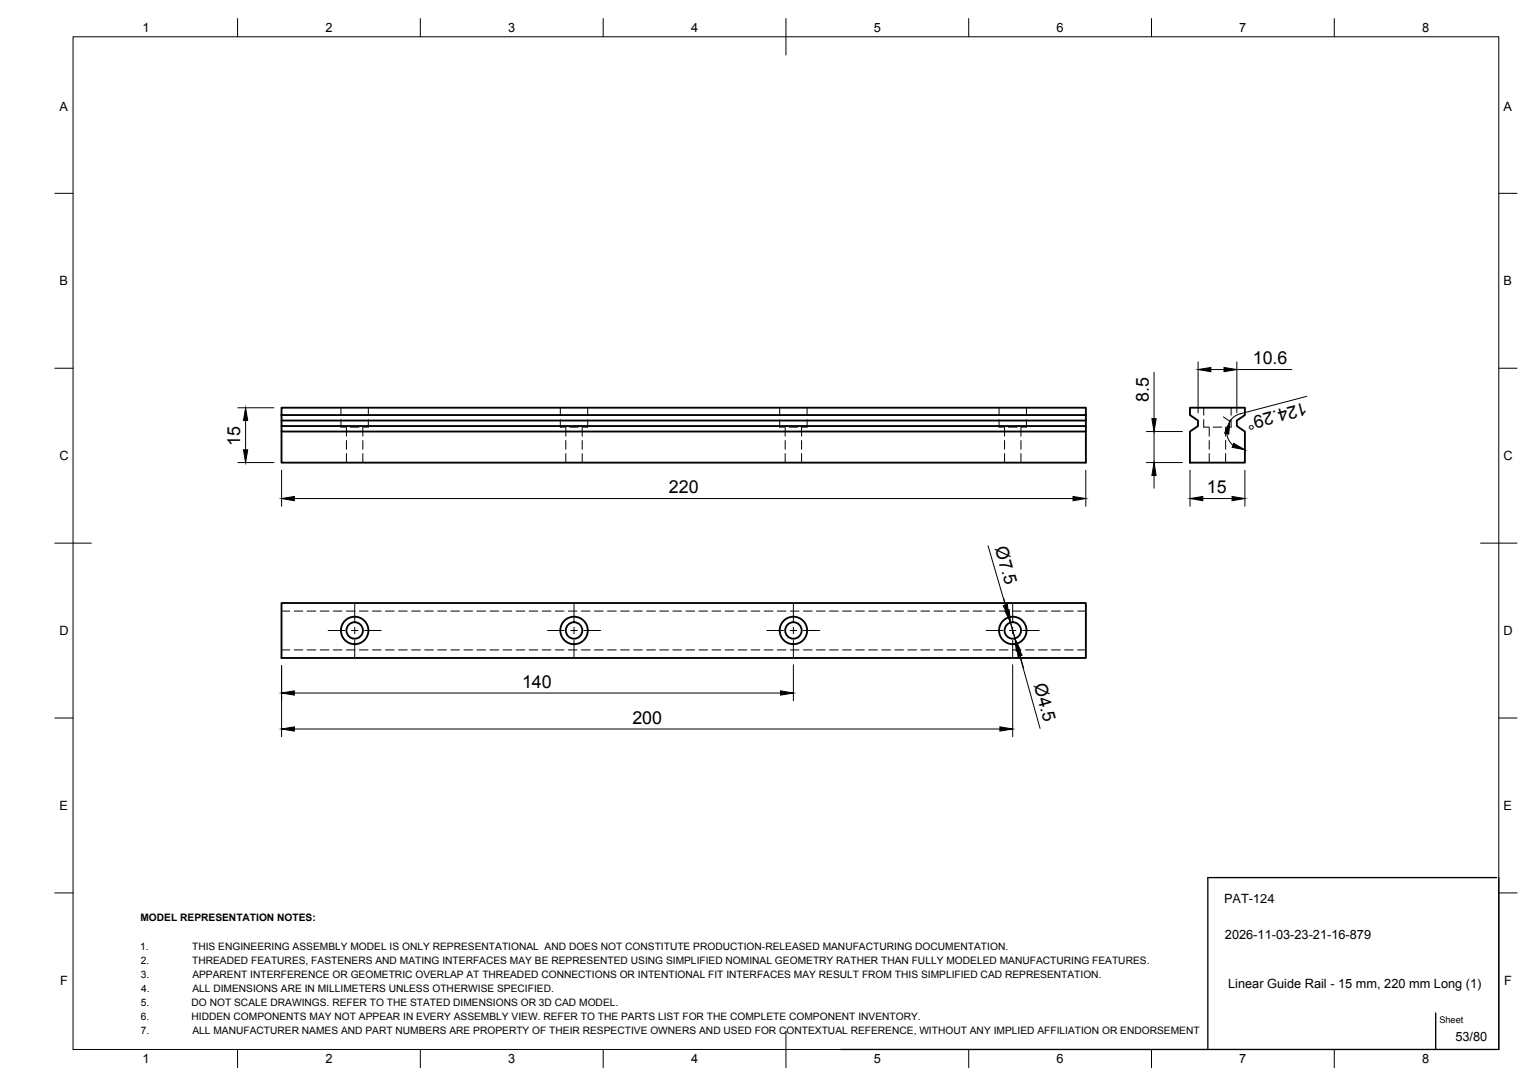
ISO-10303-21;
HEADER;
/* Generated by software containing ST-Developer
 * from STEP Tools, Inc. (www.steptools.com) 
 */

FILE_DESCRIPTION(
/* description */ ('XY cross-slide table'),
/* implementation_level */ '2;1');

FILE_NAME(
/* name */ 'Linear Guide Rail - 15 mm, 220 mm Long (1).step',
/* time_stamp */ '2026-10-28T03:22:46-07:00',
/* author */ (''),
/* organization */ (''),
/* preprocessor_version */ 'ST-DEVELOPER v20.2',
/* originating_system */ 'Autodesk Translation Framework v15.17.0.0',
/* authorisation */ '');

FILE_SCHEMA (('AUTOMOTIVE_DESIGN { 1 0 10303 214 3 1 1 }'));
ENDSEC;

DATA;
#10=MECHANICAL_DESIGN_GEOMETRIC_PRESENTATION_REPRESENTATION('',(#1735),#62984);
#1554=SHAPE_REPRESENTATION_RELATIONSHIP('SRR','None',#63409,#1637);
#1637=ADVANCED_BREP_SHAPE_REPRESENTATION('',(#1844),#62946);
#1735=STYLED_ITEM('',(#63905),#1844);
#1844=MANIFOLD_SOLID_BREP('Body1',#23033);
#2189=FACE_BOUND('',#5267,.T.);
#2190=FACE_BOUND('',#5270,.T.);
#2191=FACE_BOUND('',#5273,.T.);
#2192=FACE_BOUND('',#5276,.T.);
#2193=FACE_BOUND('',#5286,.T.);
#2194=FACE_BOUND('',#5287,.T.);
#2195=FACE_BOUND('',#5288,.T.);
#2196=FACE_BOUND('',#5289,.T.);
#2197=FACE_BOUND('',#5296,.T.);
#2198=FACE_BOUND('',#5297,.T.);
#2199=FACE_BOUND('',#5298,.T.);
#2200=FACE_BOUND('',#5299,.T.);
#2644=PLANE('',#25491);
#2645=PLANE('',#25496);
#2646=PLANE('',#25501);
#2647=PLANE('',#25506);
#2648=PLANE('',#25516);
#2649=PLANE('',#25517);
#2650=PLANE('',#25518);
#2651=PLANE('',#25519);
#2652=PLANE('',#25520);
#2653=PLANE('',#25521);
#2654=PLANE('',#25522);
#2655=PLANE('',#25523);
#2656=PLANE('',#25524);
#2657=PLANE('',#25525);
#2658=PLANE('',#25526);
#2659=PLANE('',#25527);
#2660=PLANE('',#25528);
#2661=PLANE('',#25529);
#3649=FACE_OUTER_BOUND('',#5265,.T.);
#3650=FACE_OUTER_BOUND('',#5266,.T.);
#3651=FACE_OUTER_BOUND('',#5268,.T.);
#3652=FACE_OUTER_BOUND('',#5269,.T.);
#3653=FACE_OUTER_BOUND('',#5271,.T.);
#3654=FACE_OUTER_BOUND('',#5272,.T.);
#3655=FACE_OUTER_BOUND('',#5274,.T.);
#3656=FACE_OUTER_BOUND('',#5275,.T.);
#3657=FACE_OUTER_BOUND('',#5277,.T.);
#3658=FACE_OUTER_BOUND('',#5278,.T.);
#3659=FACE_OUTER_BOUND('',#5279,.T.);
#3660=FACE_OUTER_BOUND('',#5280,.T.);
#3661=FACE_OUTER_BOUND('',#5281,.T.);
#3662=FACE_OUTER_BOUND('',#5282,.T.);
#3663=FACE_OUTER_BOUND('',#5283,.T.);
#3664=FACE_OUTER_BOUND('',#5284,.T.);
#3665=FACE_OUTER_BOUND('',#5285,.T.);
#3666=FACE_OUTER_BOUND('',#5290,.T.);
#3667=FACE_OUTER_BOUND('',#5291,.T.);
#3668=FACE_OUTER_BOUND('',#5292,.T.);
#3669=FACE_OUTER_BOUND('',#5293,.T.);
#3670=FACE_OUTER_BOUND('',#5294,.T.);
#3671=FACE_OUTER_BOUND('',#5295,.T.);
#3672=FACE_OUTER_BOUND('',#5300,.T.);
#3673=FACE_OUTER_BOUND('',#5301,.T.);
#3674=FACE_OUTER_BOUND('',#5302,.T.);
#5265=EDGE_LOOP('',(#18508,#18509,#18510,#18511));
#5266=EDGE_LOOP('',(#18512));
#5267=EDGE_LOOP('',(#18513));
#5268=EDGE_LOOP('',(#18514,#18515,#18516,#18517));
#5269=EDGE_LOOP('',(#18518));
#5270=EDGE_LOOP('',(#18519));
#5271=EDGE_LOOP('',(#18520,#18521,#18522,#18523));
#5272=EDGE_LOOP('',(#18524));
#5273=EDGE_LOOP('',(#18525));
#5274=EDGE_LOOP('',(#18526,#18527,#18528,#18529));
#5275=EDGE_LOOP('',(#18530));
#5276=EDGE_LOOP('',(#18531));
#5277=EDGE_LOOP('',(#18532,#18533,#18534,#18535));
#5278=EDGE_LOOP('',(#18536,#18537,#18538,#18539));
#5279=EDGE_LOOP('',(#18540,#18541,#18542,#18543));
#5280=EDGE_LOOP('',(#18544,#18545,#18546,#18547));
#5281=EDGE_LOOP('',(#18548,#18549,#18550,#18551));
#5282=EDGE_LOOP('',(#18552,#18553,#18554,#18555));
#5283=EDGE_LOOP('',(#18556,#18557,#18558,#18559));
#5284=EDGE_LOOP('',(#18560,#18561,#18562,#18563));
#5285=EDGE_LOOP('',(#18564,#18565,#18566,#18567));
#5286=EDGE_LOOP('',(#18568));
#5287=EDGE_LOOP('',(#18569));
#5288=EDGE_LOOP('',(#18570));
#5289=EDGE_LOOP('',(#18571));
#5290=EDGE_LOOP('',(#18572,#18573,#18574,#18575));
#5291=EDGE_LOOP('',(#18576,#18577,#18578,#18579));
#5292=EDGE_LOOP('',(#18580,#18581,#18582,#18583));
#5293=EDGE_LOOP('',(#18584,#18585,#18586,#18587));
#5294=EDGE_LOOP('',(#18588,#18589,#18590,#18591));
#5295=EDGE_LOOP('',(#18592,#18593,#18594,#18595));
#5296=EDGE_LOOP('',(#18596));
#5297=EDGE_LOOP('',(#18597));
#5298=EDGE_LOOP('',(#18598));
#5299=EDGE_LOOP('',(#18599));
#5300=EDGE_LOOP('',(#18600,#18601,#18602,#18603));
#5301=EDGE_LOOP('',(#18604,#18605,#18606,#18607,#18608,#18609,#18610,#18611,
#18612,#18613,#18614,#18615));
#5302=EDGE_LOOP('',(#18616,#18617,#18618,#18619,#18620,#18621,#18622,#18623,
#18624,#18625,#18626,#18627));
#6793=LINE('',#48410,#8280);
#6794=LINE('',#48419,#8281);
#6795=LINE('',#48428,#8282);
#6796=LINE('',#48437,#8283);
#6797=LINE('',#48445,#8284);
#6798=LINE('',#48449,#8285);
#6799=LINE('',#48453,#8286);
#6800=LINE('',#48457,#8287);
#6801=LINE('',#48461,#8288);
#6802=LINE('',#48463,#8289);
#6803=LINE('',#48465,#8290);
#6804=LINE('',#48466,#8291);
#6805=LINE('',#48469,#8292);
#6806=LINE('',#48471,#8293);
#6807=LINE('',#48472,#8294);
#6808=LINE('',#48475,#8295);
#6809=LINE('',#48477,#8296);
#6810=LINE('',#48478,#8297);
#6811=LINE('',#48481,#8298);
#6812=LINE('',#48483,#8299);
#6813=LINE('',#48484,#8300);
#6814=LINE('',#48487,#8301);
#6815=LINE('',#48489,#8302);
#6816=LINE('',#48490,#8303);
#6817=LINE('',#48493,#8304);
#6818=LINE('',#48495,#8305);
#6819=LINE('',#48496,#8306);
#6820=LINE('',#48499,#8307);
#6821=LINE('',#48501,#8308);
#6822=LINE('',#48502,#8309);
#6823=LINE('',#48505,#8310);
#6824=LINE('',#48507,#8311);
#6825=LINE('',#48508,#8312);
#6826=LINE('',#48511,#8313);
#6827=LINE('',#48513,#8314);
#6828=LINE('',#48514,#8315);
#6829=LINE('',#48517,#8316);
#6830=LINE('',#48519,#8317);
#6831=LINE('',#48520,#8318);
#6832=LINE('',#48523,#8319);
#6833=LINE('',#48525,#8320);
#6834=LINE('',#48526,#8321);
#6835=LINE('',#48528,#8322);
#6836=LINE('',#48529,#8323);
#8280=VECTOR('',#30328,0.375);
#8281=VECTOR('',#30339,0.375);
#8282=VECTOR('',#30350,0.375);
#8283=VECTOR('',#30361,0.375);
#8284=VECTOR('',#30372,0.225);
#8285=VECTOR('',#30377,0.225);
#8286=VECTOR('',#30382,0.225);
#8287=VECTOR('',#30387,0.225000000000001);
#8288=VECTOR('',#30390,1.);
#8289=VECTOR('',#30391,1.);
#8290=VECTOR('',#30392,1.);
#8291=VECTOR('',#30393,1.);
#8292=VECTOR('',#30396,1.);
#8293=VECTOR('',#30397,1.);
#8294=VECTOR('',#30398,1.);
#8295=VECTOR('',#30401,1.);
#8296=VECTOR('',#30402,1.);
#8297=VECTOR('',#30403,1.);
#8298=VECTOR('',#30406,1.);
#8299=VECTOR('',#30407,1.);
#8300=VECTOR('',#30408,1.);
#8301=VECTOR('',#30411,1.);
#8302=VECTOR('',#30412,1.);
#8303=VECTOR('',#30413,1.);
#8304=VECTOR('',#30416,1.);
#8305=VECTOR('',#30417,1.);
#8306=VECTOR('',#30418,1.);
#8307=VECTOR('',#30421,1.);
#8308=VECTOR('',#30422,1.);
#8309=VECTOR('',#30423,1.);
#8310=VECTOR('',#30426,1.);
#8311=VECTOR('',#30427,1.);
#8312=VECTOR('',#30428,1.);
#8313=VECTOR('',#30431,1.);
#8314=VECTOR('',#30432,1.);
#8315=VECTOR('',#30433,1.);
#8316=VECTOR('',#30436,1.);
#8317=VECTOR('',#30437,1.);
#8318=VECTOR('',#30438,1.);
#8319=VECTOR('',#30441,1.);
#8320=VECTOR('',#30442,1.);
#8321=VECTOR('',#30443,1.);
#8322=VECTOR('',#30446,1.);
#8323=VECTOR('',#30447,1.);
#9451=CIRCLE('',#25489,0.375);
#9452=CIRCLE('',#25490,0.375);
#9453=CIRCLE('',#25492,0.225);
#9454=CIRCLE('',#25494,0.375);
#9455=CIRCLE('',#25495,0.375);
#9456=CIRCLE('',#25497,0.225);
#9457=CIRCLE('',#25499,0.375);
#9458=CIRCLE('',#25500,0.375);
#9459=CIRCLE('',#25502,0.225);
#9460=CIRCLE('',#25504,0.375);
#9461=CIRCLE('',#25505,0.375);
#9462=CIRCLE('',#25507,0.225000000000001);
#9463=CIRCLE('',#25509,0.225);
#9464=CIRCLE('',#25511,0.225);
#9465=CIRCLE('',#25513,0.225);
#9466=CIRCLE('',#25515,0.225000000000001);
#10981=VERTEX_POINT('',#48407);
#10982=VERTEX_POINT('',#48409);
#10983=VERTEX_POINT('',#48413);
#10984=VERTEX_POINT('',#48416);
#10985=VERTEX_POINT('',#48418);
#10986=VERTEX_POINT('',#48422);
#10987=VERTEX_POINT('',#48425);
#10988=VERTEX_POINT('',#48427);
#10989=VERTEX_POINT('',#48431);
#10990=VERTEX_POINT('',#48434);
#10991=VERTEX_POINT('',#48436);
#10992=VERTEX_POINT('',#48440);
#10993=VERTEX_POINT('',#48443);
#10994=VERTEX_POINT('',#48447);
#10995=VERTEX_POINT('',#48451);
#10996=VERTEX_POINT('',#48455);
#10997=VERTEX_POINT('',#48459);
#10998=VERTEX_POINT('',#48460);
#10999=VERTEX_POINT('',#48462);
#11000=VERTEX_POINT('',#48464);
#11001=VERTEX_POINT('',#48468);
#11002=VERTEX_POINT('',#48470);
#11003=VERTEX_POINT('',#48474);
#11004=VERTEX_POINT('',#48476);
#11005=VERTEX_POINT('',#48480);
#11006=VERTEX_POINT('',#48482);
#11007=VERTEX_POINT('',#48486);
#11008=VERTEX_POINT('',#48488);
#11009=VERTEX_POINT('',#48492);
#11010=VERTEX_POINT('',#48494);
#11011=VERTEX_POINT('',#48498);
#11012=VERTEX_POINT('',#48500);
#11013=VERTEX_POINT('',#48504);
#11014=VERTEX_POINT('',#48506);
#11015=VERTEX_POINT('',#48510);
#11016=VERTEX_POINT('',#48512);
#11017=VERTEX_POINT('',#48516);
#11018=VERTEX_POINT('',#48518);
#11019=VERTEX_POINT('',#48522);
#11020=VERTEX_POINT('',#48524);
#13638=EDGE_CURVE('',#10981,#10981,#9451,.T.);
#13639=EDGE_CURVE('',#10981,#10982,#6793,.T.);
#13640=EDGE_CURVE('',#10982,#10982,#9452,.T.);
#13641=EDGE_CURVE('',#10983,#10983,#9453,.T.);
#13642=EDGE_CURVE('',#10984,#10984,#9454,.T.);
#13643=EDGE_CURVE('',#10984,#10985,#6794,.T.);
#13644=EDGE_CURVE('',#10985,#10985,#9455,.T.);
#13645=EDGE_CURVE('',#10986,#10986,#9456,.T.);
#13646=EDGE_CURVE('',#10987,#10987,#9457,.T.);
#13647=EDGE_CURVE('',#10987,#10988,#6795,.T.);
#13648=EDGE_CURVE('',#10988,#10988,#9458,.T.);
#13649=EDGE_CURVE('',#10989,#10989,#9459,.T.);
#13650=EDGE_CURVE('',#10990,#10990,#9460,.T.);
#13651=EDGE_CURVE('',#10990,#10991,#6796,.T.);
#13652=EDGE_CURVE('',#10991,#10991,#9461,.T.);
#13653=EDGE_CURVE('',#10992,#10992,#9462,.T.);
#13654=EDGE_CURVE('',#10993,#10993,#9463,.T.);
#13655=EDGE_CURVE('',#10993,#10983,#6797,.T.);
#13656=EDGE_CURVE('',#10994,#10994,#9464,.T.);
#13657=EDGE_CURVE('',#10994,#10986,#6798,.T.);
#13658=EDGE_CURVE('',#10995,#10995,#9465,.T.);
#13659=EDGE_CURVE('',#10995,#10989,#6799,.T.);
#13660=EDGE_CURVE('',#10996,#10996,#9466,.T.);
#13661=EDGE_CURVE('',#10996,#10992,#6800,.T.);
#13662=EDGE_CURVE('',#10997,#10998,#6801,.T.);
#13663=EDGE_CURVE('',#10998,#10999,#6802,.T.);
#13664=EDGE_CURVE('',#11000,#10999,#6803,.T.);
#13665=EDGE_CURVE('',#10997,#11000,#6804,.T.);
#13666=EDGE_CURVE('',#11001,#10997,#6805,.T.);
#13667=EDGE_CURVE('',#11002,#11000,#6806,.T.);
#13668=EDGE_CURVE('',#11001,#11002,#6807,.T.);
#13669=EDGE_CURVE('',#11003,#11001,#6808,.T.);
#13670=EDGE_CURVE('',#11004,#11002,#6809,.T.);
#13671=EDGE_CURVE('',#11003,#11004,#6810,.T.);
#13672=EDGE_CURVE('',#11005,#11003,#6811,.T.);
#13673=EDGE_CURVE('',#11006,#11004,#6812,.T.);
#13674=EDGE_CURVE('',#11005,#11006,#6813,.T.);
#13675=EDGE_CURVE('',#11007,#11005,#6814,.T.);
#13676=EDGE_CURVE('',#11008,#11006,#6815,.T.);
#13677=EDGE_CURVE('',#11007,#11008,#6816,.T.);
#13678=EDGE_CURVE('',#11009,#11007,#6817,.T.);
#13679=EDGE_CURVE('',#11010,#11008,#6818,.T.);
#13680=EDGE_CURVE('',#11009,#11010,#6819,.T.);
#13681=EDGE_CURVE('',#11011,#11009,#6820,.T.);
#13682=EDGE_CURVE('',#11012,#11010,#6821,.T.);
#13683=EDGE_CURVE('',#11011,#11012,#6822,.T.);
#13684=EDGE_CURVE('',#11013,#11011,#6823,.T.);
#13685=EDGE_CURVE('',#11014,#11012,#6824,.T.);
#13686=EDGE_CURVE('',#11013,#11014,#6825,.T.);
#13687=EDGE_CURVE('',#11015,#11013,#6826,.T.);
#13688=EDGE_CURVE('',#11016,#11014,#6827,.T.);
#13689=EDGE_CURVE('',#11015,#11016,#6828,.T.);
#13690=EDGE_CURVE('',#11017,#11015,#6829,.T.);
#13691=EDGE_CURVE('',#11018,#11016,#6830,.T.);
#13692=EDGE_CURVE('',#11017,#11018,#6831,.T.);
#13693=EDGE_CURVE('',#11019,#11017,#6832,.T.);
#13694=EDGE_CURVE('',#11020,#11018,#6833,.T.);
#13695=EDGE_CURVE('',#11019,#11020,#6834,.T.);
#13696=EDGE_CURVE('',#10998,#11019,#6835,.T.);
#13697=EDGE_CURVE('',#10999,#11020,#6836,.T.);
#18508=ORIENTED_EDGE('',*,*,#13638,.F.);
#18509=ORIENTED_EDGE('',*,*,#13639,.T.);
#18510=ORIENTED_EDGE('',*,*,#13640,.F.);
#18511=ORIENTED_EDGE('',*,*,#13639,.F.);
#18512=ORIENTED_EDGE('',*,*,#13638,.T.);
#18513=ORIENTED_EDGE('',*,*,#13641,.F.);
#18514=ORIENTED_EDGE('',*,*,#13642,.F.);
#18515=ORIENTED_EDGE('',*,*,#13643,.T.);
#18516=ORIENTED_EDGE('',*,*,#13644,.F.);
#18517=ORIENTED_EDGE('',*,*,#13643,.F.);
#18518=ORIENTED_EDGE('',*,*,#13642,.T.);
#18519=ORIENTED_EDGE('',*,*,#13645,.F.);
#18520=ORIENTED_EDGE('',*,*,#13646,.F.);
#18521=ORIENTED_EDGE('',*,*,#13647,.T.);
#18522=ORIENTED_EDGE('',*,*,#13648,.F.);
#18523=ORIENTED_EDGE('',*,*,#13647,.F.);
#18524=ORIENTED_EDGE('',*,*,#13646,.T.);
#18525=ORIENTED_EDGE('',*,*,#13649,.F.);
#18526=ORIENTED_EDGE('',*,*,#13650,.F.);
#18527=ORIENTED_EDGE('',*,*,#13651,.T.);
#18528=ORIENTED_EDGE('',*,*,#13652,.F.);
#18529=ORIENTED_EDGE('',*,*,#13651,.F.);
#18530=ORIENTED_EDGE('',*,*,#13650,.T.);
#18531=ORIENTED_EDGE('',*,*,#13653,.F.);
#18532=ORIENTED_EDGE('',*,*,#13654,.F.);
#18533=ORIENTED_EDGE('',*,*,#13655,.T.);
#18534=ORIENTED_EDGE('',*,*,#13641,.T.);
#18535=ORIENTED_EDGE('',*,*,#13655,.F.);
#18536=ORIENTED_EDGE('',*,*,#13656,.F.);
#18537=ORIENTED_EDGE('',*,*,#13657,.T.);
#18538=ORIENTED_EDGE('',*,*,#13645,.T.);
#18539=ORIENTED_EDGE('',*,*,#13657,.F.);
#18540=ORIENTED_EDGE('',*,*,#13658,.F.);
#18541=ORIENTED_EDGE('',*,*,#13659,.T.);
#18542=ORIENTED_EDGE('',*,*,#13649,.T.);
#18543=ORIENTED_EDGE('',*,*,#13659,.F.);
#18544=ORIENTED_EDGE('',*,*,#13660,.F.);
#18545=ORIENTED_EDGE('',*,*,#13661,.T.);
#18546=ORIENTED_EDGE('',*,*,#13653,.T.);
#18547=ORIENTED_EDGE('',*,*,#13661,.F.);
#18548=ORIENTED_EDGE('',*,*,#13662,.T.);
#18549=ORIENTED_EDGE('',*,*,#13663,.T.);
#18550=ORIENTED_EDGE('',*,*,#13664,.F.);
#18551=ORIENTED_EDGE('',*,*,#13665,.F.);
#18552=ORIENTED_EDGE('',*,*,#13666,.T.);
#18553=ORIENTED_EDGE('',*,*,#13665,.T.);
#18554=ORIENTED_EDGE('',*,*,#13667,.F.);
#18555=ORIENTED_EDGE('',*,*,#13668,.F.);
#18556=ORIENTED_EDGE('',*,*,#13669,.T.);
#18557=ORIENTED_EDGE('',*,*,#13668,.T.);
#18558=ORIENTED_EDGE('',*,*,#13670,.F.);
#18559=ORIENTED_EDGE('',*,*,#13671,.F.);
#18560=ORIENTED_EDGE('',*,*,#13672,.T.);
#18561=ORIENTED_EDGE('',*,*,#13671,.T.);
#18562=ORIENTED_EDGE('',*,*,#13673,.F.);
#18563=ORIENTED_EDGE('',*,*,#13674,.F.);
#18564=ORIENTED_EDGE('',*,*,#13675,.T.);
#18565=ORIENTED_EDGE('',*,*,#13674,.T.);
#18566=ORIENTED_EDGE('',*,*,#13676,.F.);
#18567=ORIENTED_EDGE('',*,*,#13677,.F.);
#18568=ORIENTED_EDGE('',*,*,#13652,.T.);
#18569=ORIENTED_EDGE('',*,*,#13648,.T.);
#18570=ORIENTED_EDGE('',*,*,#13644,.T.);
#18571=ORIENTED_EDGE('',*,*,#13640,.T.);
#18572=ORIENTED_EDGE('',*,*,#13678,.T.);
#18573=ORIENTED_EDGE('',*,*,#13677,.T.);
#18574=ORIENTED_EDGE('',*,*,#13679,.F.);
#18575=ORIENTED_EDGE('',*,*,#13680,.F.);
#18576=ORIENTED_EDGE('',*,*,#13681,.T.);
#18577=ORIENTED_EDGE('',*,*,#13680,.T.);
#18578=ORIENTED_EDGE('',*,*,#13682,.F.);
#18579=ORIENTED_EDGE('',*,*,#13683,.F.);
#18580=ORIENTED_EDGE('',*,*,#13684,.T.);
#18581=ORIENTED_EDGE('',*,*,#13683,.T.);
#18582=ORIENTED_EDGE('',*,*,#13685,.F.);
#18583=ORIENTED_EDGE('',*,*,#13686,.F.);
#18584=ORIENTED_EDGE('',*,*,#13687,.T.);
#18585=ORIENTED_EDGE('',*,*,#13686,.T.);
#18586=ORIENTED_EDGE('',*,*,#13688,.F.);
#18587=ORIENTED_EDGE('',*,*,#13689,.F.);
#18588=ORIENTED_EDGE('',*,*,#13690,.T.);
#18589=ORIENTED_EDGE('',*,*,#13689,.T.);
#18590=ORIENTED_EDGE('',*,*,#13691,.F.);
#18591=ORIENTED_EDGE('',*,*,#13692,.F.);
#18592=ORIENTED_EDGE('',*,*,#13693,.T.);
#18593=ORIENTED_EDGE('',*,*,#13692,.T.);
#18594=ORIENTED_EDGE('',*,*,#13694,.F.);
#18595=ORIENTED_EDGE('',*,*,#13695,.F.);
#18596=ORIENTED_EDGE('',*,*,#13654,.T.);
#18597=ORIENTED_EDGE('',*,*,#13656,.T.);
#18598=ORIENTED_EDGE('',*,*,#13658,.T.);
#18599=ORIENTED_EDGE('',*,*,#13660,.T.);
#18600=ORIENTED_EDGE('',*,*,#13696,.T.);
#18601=ORIENTED_EDGE('',*,*,#13695,.T.);
#18602=ORIENTED_EDGE('',*,*,#13697,.F.);
#18603=ORIENTED_EDGE('',*,*,#13663,.F.);
#18604=ORIENTED_EDGE('',*,*,#13697,.T.);
#18605=ORIENTED_EDGE('',*,*,#13694,.T.);
#18606=ORIENTED_EDGE('',*,*,#13691,.T.);
#18607=ORIENTED_EDGE('',*,*,#13688,.T.);
#18608=ORIENTED_EDGE('',*,*,#13685,.T.);
#18609=ORIENTED_EDGE('',*,*,#13682,.T.);
#18610=ORIENTED_EDGE('',*,*,#13679,.T.);
#18611=ORIENTED_EDGE('',*,*,#13676,.T.);
#18612=ORIENTED_EDGE('',*,*,#13673,.T.);
#18613=ORIENTED_EDGE('',*,*,#13670,.T.);
#18614=ORIENTED_EDGE('',*,*,#13667,.T.);
#18615=ORIENTED_EDGE('',*,*,#13664,.T.);
#18616=ORIENTED_EDGE('',*,*,#13696,.F.);
#18617=ORIENTED_EDGE('',*,*,#13662,.F.);
#18618=ORIENTED_EDGE('',*,*,#13666,.F.);
#18619=ORIENTED_EDGE('',*,*,#13669,.F.);
#18620=ORIENTED_EDGE('',*,*,#13672,.F.);
#18621=ORIENTED_EDGE('',*,*,#13675,.F.);
#18622=ORIENTED_EDGE('',*,*,#13678,.F.);
#18623=ORIENTED_EDGE('',*,*,#13681,.F.);
#18624=ORIENTED_EDGE('',*,*,#13684,.F.);
#18625=ORIENTED_EDGE('',*,*,#13687,.F.);
#18626=ORIENTED_EDGE('',*,*,#13690,.F.);
#18627=ORIENTED_EDGE('',*,*,#13693,.F.);
#21408=CYLINDRICAL_SURFACE('',#25488,0.375);
#21409=CYLINDRICAL_SURFACE('',#25493,0.375);
#21410=CYLINDRICAL_SURFACE('',#25498,0.375);
#21411=CYLINDRICAL_SURFACE('',#25503,0.375);
#21412=CYLINDRICAL_SURFACE('',#25508,0.225);
#21413=CYLINDRICAL_SURFACE('',#25510,0.225);
#21414=CYLINDRICAL_SURFACE('',#25512,0.225);
#21415=CYLINDRICAL_SURFACE('',#25514,0.225000000000001);
#22430=ADVANCED_FACE('',(#3649),#21408,.F.);
#22431=ADVANCED_FACE('',(#3650,#2189),#2644,.T.);
#22432=ADVANCED_FACE('',(#3651),#21409,.F.);
#22433=ADVANCED_FACE('',(#3652,#2190),#2645,.T.);
#22434=ADVANCED_FACE('',(#3653),#21410,.F.);
#22435=ADVANCED_FACE('',(#3654,#2191),#2646,.T.);
#22436=ADVANCED_FACE('',(#3655),#21411,.F.);
#22437=ADVANCED_FACE('',(#3656,#2192),#2647,.T.);
#22438=ADVANCED_FACE('',(#3657),#21412,.F.);
#22439=ADVANCED_FACE('',(#3658),#21413,.F.);
#22440=ADVANCED_FACE('',(#3659),#21414,.F.);
#22441=ADVANCED_FACE('',(#3660),#21415,.F.);
#22442=ADVANCED_FACE('',(#3661),#2648,.T.);
#22443=ADVANCED_FACE('',(#3662),#2649,.T.);
#22444=ADVANCED_FACE('',(#3663),#2650,.T.);
#22445=ADVANCED_FACE('',(#3664),#2651,.T.);
#22446=ADVANCED_FACE('',(#3665,#2193,#2194,#2195,#2196),#2652,.T.);
#22447=ADVANCED_FACE('',(#3666),#2653,.T.);
#22448=ADVANCED_FACE('',(#3667),#2654,.T.);
#22449=ADVANCED_FACE('',(#3668),#2655,.T.);
#22450=ADVANCED_FACE('',(#3669),#2656,.T.);
#22451=ADVANCED_FACE('',(#3670),#2657,.T.);
#22452=ADVANCED_FACE('',(#3671,#2197,#2198,#2199,#2200),#2658,.T.);
#22453=ADVANCED_FACE('',(#3672),#2659,.T.);
#22454=ADVANCED_FACE('',(#3673),#2660,.T.);
#22455=ADVANCED_FACE('',(#3674),#2661,.F.);
#23033=CLOSED_SHELL('',(#22430,#22431,#22432,#22433,#22434,#22435,#22436,
#22437,#22438,#22439,#22440,#22441,#22442,#22443,#22444,#22445,#22446,#22447,
#22448,#22449,#22450,#22451,#22452,#22453,#22454,#22455));
#25487=AXIS2_PLACEMENT_3D('',#48405,#30322,#30323);
#25488=AXIS2_PLACEMENT_3D('',#48406,#30324,#30325);
#25489=AXIS2_PLACEMENT_3D('',#48408,#30326,#30327);
#25490=AXIS2_PLACEMENT_3D('',#48411,#30329,#30330);
#25491=AXIS2_PLACEMENT_3D('',#48412,#30331,#30332);
#25492=AXIS2_PLACEMENT_3D('',#48414,#30333,#30334);
#25493=AXIS2_PLACEMENT_3D('',#48415,#30335,#30336);
#25494=AXIS2_PLACEMENT_3D('',#48417,#30337,#30338);
#25495=AXIS2_PLACEMENT_3D('',#48420,#30340,#30341);
#25496=AXIS2_PLACEMENT_3D('',#48421,#30342,#30343);
#25497=AXIS2_PLACEMENT_3D('',#48423,#30344,#30345);
#25498=AXIS2_PLACEMENT_3D('',#48424,#30346,#30347);
#25499=AXIS2_PLACEMENT_3D('',#48426,#30348,#30349);
#25500=AXIS2_PLACEMENT_3D('',#48429,#30351,#30352);
#25501=AXIS2_PLACEMENT_3D('',#48430,#30353,#30354);
#25502=AXIS2_PLACEMENT_3D('',#48432,#30355,#30356);
#25503=AXIS2_PLACEMENT_3D('',#48433,#30357,#30358);
#25504=AXIS2_PLACEMENT_3D('',#48435,#30359,#30360);
#25505=AXIS2_PLACEMENT_3D('',#48438,#30362,#30363);
#25506=AXIS2_PLACEMENT_3D('',#48439,#30364,#30365);
#25507=AXIS2_PLACEMENT_3D('',#48441,#30366,#30367);
#25508=AXIS2_PLACEMENT_3D('',#48442,#30368,#30369);
#25509=AXIS2_PLACEMENT_3D('',#48444,#30370,#30371);
#25510=AXIS2_PLACEMENT_3D('',#48446,#30373,#30374);
#25511=AXIS2_PLACEMENT_3D('',#48448,#30375,#30376);
#25512=AXIS2_PLACEMENT_3D('',#48450,#30378,#30379);
#25513=AXIS2_PLACEMENT_3D('',#48452,#30380,#30381);
#25514=AXIS2_PLACEMENT_3D('',#48454,#30383,#30384);
#25515=AXIS2_PLACEMENT_3D('',#48456,#30385,#30386);
#25516=AXIS2_PLACEMENT_3D('',#48458,#30388,#30389);
#25517=AXIS2_PLACEMENT_3D('',#48467,#30394,#30395);
#25518=AXIS2_PLACEMENT_3D('',#48473,#30399,#30400);
#25519=AXIS2_PLACEMENT_3D('',#48479,#30404,#30405);
#25520=AXIS2_PLACEMENT_3D('',#48485,#30409,#30410);
#25521=AXIS2_PLACEMENT_3D('',#48491,#30414,#30415);
#25522=AXIS2_PLACEMENT_3D('',#48497,#30419,#30420);
#25523=AXIS2_PLACEMENT_3D('',#48503,#30424,#30425);
#25524=AXIS2_PLACEMENT_3D('',#48509,#30429,#30430);
#25525=AXIS2_PLACEMENT_3D('',#48515,#30434,#30435);
#25526=AXIS2_PLACEMENT_3D('',#48521,#30439,#30440);
#25527=AXIS2_PLACEMENT_3D('',#48527,#30444,#30445);
#25528=AXIS2_PLACEMENT_3D('',#48530,#30448,#30449);
#25529=AXIS2_PLACEMENT_3D('',#48531,#30450,#30451);
#30322=DIRECTION('axis',(0.,0.,1.));
#30323=DIRECTION('refdir',(1.,0.,0.));
#30324=DIRECTION('center_axis',(0.,0.,1.));
#30325=DIRECTION('ref_axis',(1.,0.,0.));
#30326=DIRECTION('center_axis',(0.,0.,1.));
#30327=DIRECTION('ref_axis',(1.,0.,0.));
#30328=DIRECTION('',(0.,0.,1.));
#30329=DIRECTION('center_axis',(0.,0.,-1.));
#30330=DIRECTION('ref_axis',(1.,0.,0.));
#30331=DIRECTION('center_axis',(0.,0.,1.));
#30332=DIRECTION('ref_axis',(1.,0.,0.));
#30333=DIRECTION('center_axis',(0.,0.,1.));
#30334=DIRECTION('ref_axis',(1.,0.,0.));
#30335=DIRECTION('center_axis',(0.,0.,1.));
#30336=DIRECTION('ref_axis',(1.,0.,0.));
#30337=DIRECTION('center_axis',(0.,0.,1.));
#30338=DIRECTION('ref_axis',(1.,0.,0.));
#30339=DIRECTION('',(0.,0.,1.));
#30340=DIRECTION('center_axis',(0.,0.,-1.));
#30341=DIRECTION('ref_axis',(1.,0.,0.));
#30342=DIRECTION('center_axis',(0.,0.,1.));
#30343=DIRECTION('ref_axis',(1.,0.,0.));
#30344=DIRECTION('center_axis',(0.,0.,1.));
#30345=DIRECTION('ref_axis',(1.,0.,0.));
#30346=DIRECTION('center_axis',(0.,0.,1.));
#30347=DIRECTION('ref_axis',(1.,0.,0.));
#30348=DIRECTION('center_axis',(0.,0.,1.));
#30349=DIRECTION('ref_axis',(1.,0.,0.));
#30350=DIRECTION('',(0.,0.,1.));
#30351=DIRECTION('center_axis',(0.,0.,-1.));
#30352=DIRECTION('ref_axis',(1.,0.,0.));
#30353=DIRECTION('center_axis',(0.,0.,1.));
#30354=DIRECTION('ref_axis',(1.,0.,0.));
#30355=DIRECTION('center_axis',(0.,0.,1.));
#30356=DIRECTION('ref_axis',(1.,0.,0.));
#30357=DIRECTION('center_axis',(0.,0.,1.));
#30358=DIRECTION('ref_axis',(1.,0.,0.));
#30359=DIRECTION('center_axis',(0.,0.,1.));
#30360=DIRECTION('ref_axis',(1.,0.,0.));
#30361=DIRECTION('',(0.,0.,1.));
#30362=DIRECTION('center_axis',(0.,0.,-1.));
#30363=DIRECTION('ref_axis',(1.,0.,0.));
#30364=DIRECTION('center_axis',(0.,0.,1.));
#30365=DIRECTION('ref_axis',(1.,0.,0.));
#30366=DIRECTION('center_axis',(0.,0.,1.));
#30367=DIRECTION('ref_axis',(1.,0.,0.));
#30368=DIRECTION('center_axis',(0.,0.,1.));
#30369=DIRECTION('ref_axis',(1.,0.,0.));
#30370=DIRECTION('center_axis',(0.,0.,1.));
#30371=DIRECTION('ref_axis',(1.,0.,0.));
#30372=DIRECTION('',(0.,0.,1.));
#30373=DIRECTION('center_axis',(0.,0.,1.));
#30374=DIRECTION('ref_axis',(1.,0.,0.));
#30375=DIRECTION('center_axis',(0.,0.,1.));
#30376=DIRECTION('ref_axis',(1.,0.,0.));
#30377=DIRECTION('',(0.,0.,1.));
#30378=DIRECTION('center_axis',(0.,0.,1.));
#30379=DIRECTION('ref_axis',(1.,0.,0.));
#30380=DIRECTION('center_axis',(0.,0.,1.));
#30381=DIRECTION('ref_axis',(1.,0.,0.));
#30382=DIRECTION('',(0.,0.,1.));
#30383=DIRECTION('center_axis',(0.,0.,1.));
#30384=DIRECTION('ref_axis',(1.,0.,0.));
#30385=DIRECTION('center_axis',(0.,0.,1.));
#30386=DIRECTION('ref_axis',(1.,0.,0.));
#30387=DIRECTION('',(0.,0.,1.));
#30388=DIRECTION('center_axis',(0.,-0.56333682464151,0.826227342807548));
#30389=DIRECTION('ref_axis',(0.,-0.826227342807548,-0.56333682464151));
#30390=DIRECTION('',(0.,-0.826227342807548,-0.56333682464151));
#30391=DIRECTION('',(1.,0.,0.));
#30392=DIRECTION('',(0.,-0.826227342807548,-0.56333682464151));
#30393=DIRECTION('',(1.,0.,0.));
#30394=DIRECTION('center_axis',(0.,-1.,0.));
#30395=DIRECTION('ref_axis',(0.,0.,-1.));
#30396=DIRECTION('',(0.,0.,-1.));
#30397=DIRECTION('',(0.,0.,-1.));
#30398=DIRECTION('',(1.,0.,0.));
#30399=DIRECTION('center_axis',(0.,-0.56333682464151,-0.826227342807548));
#30400=DIRECTION('ref_axis',(0.,0.826227342807548,-0.56333682464151));
#30401=DIRECTION('',(0.,0.826227342807548,-0.56333682464151));
#30402=DIRECTION('',(0.,0.826227342807548,-0.56333682464151));
#30403=DIRECTION('',(1.,0.,0.));
#30404=DIRECTION('center_axis',(0.,-1.,0.));
#30405=DIRECTION('ref_axis',(0.,0.,-1.));
#30406=DIRECTION('',(0.,0.,-1.));
#30407=DIRECTION('',(0.,0.,-1.));
#30408=DIRECTION('',(1.,0.,0.));
#30409=DIRECTION('center_axis',(0.,0.,1.));
#30410=DIRECTION('ref_axis',(0.,-1.,0.));
#30411=DIRECTION('',(0.,-1.,0.));
#30412=DIRECTION('',(0.,-1.,0.));
#30413=DIRECTION('',(1.,0.,0.));
#30414=DIRECTION('center_axis',(0.,1.,0.));
#30415=DIRECTION('ref_axis',(0.,0.,1.));
#30416=DIRECTION('',(0.,0.,1.));
#30417=DIRECTION('',(0.,0.,1.));
#30418=DIRECTION('',(1.,0.,0.));
#30419=DIRECTION('center_axis',(0.,0.56333682464151,-0.826227342807548));
#30420=DIRECTION('ref_axis',(0.,0.826227342807548,0.56333682464151));
#30421=DIRECTION('',(0.,0.826227342807548,0.56333682464151));
#30422=DIRECTION('',(0.,0.826227342807548,0.56333682464151));
#30423=DIRECTION('',(1.,0.,0.));
#30424=DIRECTION('center_axis',(0.,1.,0.));
#30425=DIRECTION('ref_axis',(0.,0.,1.));
#30426=DIRECTION('',(0.,0.,1.));
#30427=DIRECTION('',(0.,0.,1.));
#30428=DIRECTION('',(1.,0.,0.));
#30429=DIRECTION('center_axis',(0.,0.56333682464151,0.826227342807548));
#30430=DIRECTION('ref_axis',(0.,-0.826227342807548,0.56333682464151));
#30431=DIRECTION('',(0.,-0.826227342807548,0.56333682464151));
#30432=DIRECTION('',(0.,-0.826227342807548,0.56333682464151));
#30433=DIRECTION('',(1.,0.,0.));
#30434=DIRECTION('center_axis',(0.,1.,0.));
#30435=DIRECTION('ref_axis',(0.,0.,1.));
#30436=DIRECTION('',(0.,0.,1.));
#30437=DIRECTION('',(0.,0.,1.));
#30438=DIRECTION('',(1.,0.,0.));
#30439=DIRECTION('center_axis',(0.,0.,-1.));
#30440=DIRECTION('ref_axis',(0.,1.,0.));
#30441=DIRECTION('',(0.,1.,0.));
#30442=DIRECTION('',(0.,1.,0.));
#30443=DIRECTION('',(1.,0.,0.));
#30444=DIRECTION('center_axis',(0.,-1.,0.));
#30445=DIRECTION('ref_axis',(0.,0.,-1.));
#30446=DIRECTION('',(0.,0.,-1.));
#30447=DIRECTION('',(0.,0.,-1.));
#30448=DIRECTION('center_axis',(1.,0.,0.));
#30449=DIRECTION('ref_axis',(0.,0.,-1.));
#30450=DIRECTION('center_axis',(1.,0.,0.));
#30451=DIRECTION('ref_axis',(0.,0.,-1.));
#48405=CARTESIAN_POINT('',(0.,0.,0.));
#48406=CARTESIAN_POINT('Origin',(14.,0.,0.97));
#48407=CARTESIAN_POINT('',(13.625,-4.59242549680257E-17,0.97));
#48408=CARTESIAN_POINT('Origin',(14.,0.,0.97));
#48409=CARTESIAN_POINT('',(13.625,4.59242549680257E-17,1.5));
#48410=CARTESIAN_POINT('',(13.625,-4.59242549680257E-17,0.97));
#48411=CARTESIAN_POINT('Origin',(14.,0.,1.5));
#48412=CARTESIAN_POINT('Origin',(14.,0.,0.97));
#48413=CARTESIAN_POINT('',(13.775,-2.75545529808154E-17,0.97));
#48414=CARTESIAN_POINT('Origin',(14.,0.,0.97));
#48415=CARTESIAN_POINT('Origin',(8.,0.,0.97));
#48416=CARTESIAN_POINT('',(7.625,-4.59242549680257E-17,0.97));
#48417=CARTESIAN_POINT('Origin',(8.,0.,0.97));
#48418=CARTESIAN_POINT('',(7.625,4.59242549680257E-17,1.5));
#48419=CARTESIAN_POINT('',(7.625,-4.59242549680257E-17,0.97));
#48420=CARTESIAN_POINT('Origin',(8.,0.,1.5));
#48421=CARTESIAN_POINT('Origin',(8.,0.,0.97));
#48422=CARTESIAN_POINT('',(7.775,-2.75545529808154E-17,0.97));
#48423=CARTESIAN_POINT('Origin',(8.,0.,0.97));
#48424=CARTESIAN_POINT('Origin',(2.,0.,0.97));
#48425=CARTESIAN_POINT('',(1.625,-4.59242549680257E-17,0.97));
#48426=CARTESIAN_POINT('Origin',(2.,0.,0.97));
#48427=CARTESIAN_POINT('',(1.625,4.59242549680257E-17,1.5));
#48428=CARTESIAN_POINT('',(1.625,-4.59242549680257E-17,0.97));
#48429=CARTESIAN_POINT('Origin',(2.,0.,1.5));
#48430=CARTESIAN_POINT('Origin',(2.,0.,0.97));
#48431=CARTESIAN_POINT('',(1.775,-2.75545529808155E-17,0.97));
#48432=CARTESIAN_POINT('Origin',(2.,0.,0.97));
#48433=CARTESIAN_POINT('Origin',(20.,0.,0.97));
#48434=CARTESIAN_POINT('',(19.625,-4.59242549680257E-17,0.97));
#48435=CARTESIAN_POINT('Origin',(20.,0.,0.97));
#48436=CARTESIAN_POINT('',(19.625,4.59242549680257E-17,1.5));
#48437=CARTESIAN_POINT('',(19.625,-4.59242549680257E-17,0.97));
#48438=CARTESIAN_POINT('Origin',(20.,0.,1.5));
#48439=CARTESIAN_POINT('Origin',(20.,0.,0.97));
#48440=CARTESIAN_POINT('',(19.775,-2.75545529808156E-17,0.97));
#48441=CARTESIAN_POINT('Origin',(20.,0.,0.97));
#48442=CARTESIAN_POINT('Origin',(14.,0.,-0.1));
#48443=CARTESIAN_POINT('',(13.775,-2.75545529808154E-17,0.));
#48444=CARTESIAN_POINT('Origin',(14.,0.,0.));
#48445=CARTESIAN_POINT('',(13.775,-2.75545529808154E-17,-0.1));
#48446=CARTESIAN_POINT('Origin',(8.,0.,-0.1));
#48447=CARTESIAN_POINT('',(7.775,-2.75545529808154E-17,0.));
#48448=CARTESIAN_POINT('Origin',(8.,0.,0.));
#48449=CARTESIAN_POINT('',(7.775,-2.75545529808154E-17,-0.1));
#48450=CARTESIAN_POINT('Origin',(2.,0.,-0.1));
#48451=CARTESIAN_POINT('',(1.775,-2.75545529808155E-17,0.));
#48452=CARTESIAN_POINT('Origin',(2.,0.,0.));
#48453=CARTESIAN_POINT('',(1.775,-2.75545529808155E-17,-0.1));
#48454=CARTESIAN_POINT('Origin',(20.,0.,-0.1));
#48455=CARTESIAN_POINT('',(19.775,-2.75545529808156E-17,0.));
#48456=CARTESIAN_POINT('Origin',(20.,0.,0.));
#48457=CARTESIAN_POINT('',(19.775,-2.75545529808156E-17,-0.1));
#48458=CARTESIAN_POINT('Origin',(0.,-0.53,1.));
#48459=CARTESIAN_POINT('',(0.,-0.53,1.));
#48460=CARTESIAN_POINT('',(0.,-0.75,0.85));
#48461=CARTESIAN_POINT('',(0.,-0.53,1.));
#48462=CARTESIAN_POINT('',(22.,-0.75,0.85));
#48463=CARTESIAN_POINT('',(0.,-0.75,0.85));
#48464=CARTESIAN_POINT('',(22.,-0.53,1.));
#48465=CARTESIAN_POINT('',(22.,-0.53,1.));
#48466=CARTESIAN_POINT('',(0.,-0.53,1.));
#48467=CARTESIAN_POINT('Origin',(0.,-0.53,1.15));
#48468=CARTESIAN_POINT('',(0.,-0.53,1.15));
#48469=CARTESIAN_POINT('',(0.,-0.53,1.15));
#48470=CARTESIAN_POINT('',(22.,-0.53,1.15));
#48471=CARTESIAN_POINT('',(22.,-0.53,1.15));
#48472=CARTESIAN_POINT('',(0.,-0.53,1.15));
#48473=CARTESIAN_POINT('Origin',(0.,-0.75,1.3));
#48474=CARTESIAN_POINT('',(0.,-0.75,1.3));
#48475=CARTESIAN_POINT('',(0.,-0.75,1.3));
#48476=CARTESIAN_POINT('',(22.,-0.75,1.3));
#48477=CARTESIAN_POINT('',(22.,-0.75,1.3));
#48478=CARTESIAN_POINT('',(0.,-0.75,1.3));
#48479=CARTESIAN_POINT('Origin',(0.,-0.75,1.5));
#48480=CARTESIAN_POINT('',(0.,-0.75,1.5));
#48481=CARTESIAN_POINT('',(0.,-0.75,1.5));
#48482=CARTESIAN_POINT('',(22.,-0.75,1.5));
#48483=CARTESIAN_POINT('',(22.,-0.75,1.5));
#48484=CARTESIAN_POINT('',(0.,-0.75,1.5));
#48485=CARTESIAN_POINT('Origin',(0.,0.75,1.5));
#48486=CARTESIAN_POINT('',(0.,0.75,1.5));
#48487=CARTESIAN_POINT('',(0.,0.75,1.5));
#48488=CARTESIAN_POINT('',(22.,0.75,1.5));
#48489=CARTESIAN_POINT('',(22.,0.75,1.5));
#48490=CARTESIAN_POINT('',(0.,0.75,1.5));
#48491=CARTESIAN_POINT('Origin',(0.,0.75,1.3));
#48492=CARTESIAN_POINT('',(0.,0.75,1.3));
#48493=CARTESIAN_POINT('',(0.,0.75,1.3));
#48494=CARTESIAN_POINT('',(22.,0.75,1.3));
#48495=CARTESIAN_POINT('',(22.,0.75,1.3));
#48496=CARTESIAN_POINT('',(0.,0.75,1.3));
#48497=CARTESIAN_POINT('Origin',(0.,0.53,1.15));
#48498=CARTESIAN_POINT('',(0.,0.53,1.15));
#48499=CARTESIAN_POINT('',(0.,0.53,1.15));
#48500=CARTESIAN_POINT('',(22.,0.53,1.15));
#48501=CARTESIAN_POINT('',(22.,0.53,1.15));
#48502=CARTESIAN_POINT('',(0.,0.53,1.15));
#48503=CARTESIAN_POINT('Origin',(0.,0.53,1.));
#48504=CARTESIAN_POINT('',(0.,0.53,1.));
#48505=CARTESIAN_POINT('',(0.,0.53,1.));
#48506=CARTESIAN_POINT('',(22.,0.53,1.));
#48507=CARTESIAN_POINT('',(22.,0.53,1.));
#48508=CARTESIAN_POINT('',(0.,0.53,1.));
#48509=CARTESIAN_POINT('Origin',(0.,0.75,0.85));
#48510=CARTESIAN_POINT('',(0.,0.75,0.85));
#48511=CARTESIAN_POINT('',(0.,0.75,0.85));
#48512=CARTESIAN_POINT('',(22.,0.75,0.85));
#48513=CARTESIAN_POINT('',(22.,0.75,0.85));
#48514=CARTESIAN_POINT('',(0.,0.75,0.85));
#48515=CARTESIAN_POINT('Origin',(0.,0.75,0.));
#48516=CARTESIAN_POINT('',(0.,0.75,0.));
#48517=CARTESIAN_POINT('',(0.,0.75,0.));
#48518=CARTESIAN_POINT('',(22.,0.75,0.));
#48519=CARTESIAN_POINT('',(22.,0.75,0.));
#48520=CARTESIAN_POINT('',(0.,0.75,0.));
#48521=CARTESIAN_POINT('Origin',(0.,-0.75,0.));
#48522=CARTESIAN_POINT('',(0.,-0.75,0.));
#48523=CARTESIAN_POINT('',(0.,-0.75,0.));
#48524=CARTESIAN_POINT('',(22.,-0.75,0.));
#48525=CARTESIAN_POINT('',(22.,-0.75,0.));
#48526=CARTESIAN_POINT('',(0.,-0.75,0.));
#48527=CARTESIAN_POINT('Origin',(0.,-0.75,0.85));
#48528=CARTESIAN_POINT('',(0.,-0.75,0.85));
#48529=CARTESIAN_POINT('',(22.,-0.75,0.85));
#48530=CARTESIAN_POINT('Origin',(22.,0.,0.75));
#48531=CARTESIAN_POINT('Origin',(0.,0.,0.75));
#62847=UNCERTAINTY_MEASURE_WITH_UNIT(LENGTH_MEASURE(0.001),#62985,
'DISTANCE_ACCURACY_VALUE',
'Maximum model space distance between geometric entities at asserted c
onnectivities');
#62885=UNCERTAINTY_MEASURE_WITH_UNIT(LENGTH_MEASURE(0.001),#62985,
'DISTANCE_ACCURACY_VALUE',
'Maximum model space distance between geometric entities at asserted c
onnectivities');
#62946=(
GEOMETRIC_REPRESENTATION_CONTEXT(3)
GLOBAL_UNCERTAINTY_ASSIGNED_CONTEXT((#62847))
GLOBAL_UNIT_ASSIGNED_CONTEXT((#62985,#62987,#62988))
REPRESENTATION_CONTEXT('','3D')
);
#62984=(
GEOMETRIC_REPRESENTATION_CONTEXT(3)
GLOBAL_UNCERTAINTY_ASSIGNED_CONTEXT((#62885))
GLOBAL_UNIT_ASSIGNED_CONTEXT((#62985,#62987,#62988))
REPRESENTATION_CONTEXT('','3D')
);
#62985=(
LENGTH_UNIT()
NAMED_UNIT(*)
SI_UNIT(.CENTI.,.METRE.)
);
#62987=(
NAMED_UNIT(*)
PLANE_ANGLE_UNIT()
SI_UNIT($,.RADIAN.)
);
#62988=(
NAMED_UNIT(*)
SI_UNIT($,.STERADIAN.)
SOLID_ANGLE_UNIT()
);
#63049=SHAPE_DEFINITION_REPRESENTATION(#63227,#63409);
#63227=PRODUCT_DEFINITION_SHAPE('',$,#63508);
#63409=SHAPE_REPRESENTATION('',(#25487),#62946);
#63447=PRODUCT_DEFINITION_CONTEXT('part definition',#63743,'design');
#63508=PRODUCT_DEFINITION('Linear Guide Rail - 15 mm, 220 mm Long (1)',
'Linear Guide Rail - 15 mm, 220 mm Long (1)',#63606,#63447);
#63606=PRODUCT_DEFINITION_FORMATION('',$,#63805);
#63743=APPLICATION_CONTEXT(
'Core Data for Automotive Mechanical Design Process');
#63744=PRODUCT_CONTEXT('part definition',#63743,'mechanical');
#63805=PRODUCT('Linear Guide Rail - 15 mm, 220 mm Long (1)',
'Linear Guide Rail - 15 mm, 220 mm Long (1)',
'Linear Guide Rail - 15 mm, 220 mm Long (1)',(#63744));
#63899=COLOUR_RGB('Sky Blue',0.24,0.69,0.87);
#63900=FILL_AREA_STYLE_COLOUR('',#63899);
#63901=FILL_AREA_STYLE('',(#63900));
#63902=SURFACE_STYLE_FILL_AREA(#63901);
#63903=SURFACE_SIDE_STYLE('',(#63902));
#63904=SURFACE_STYLE_USAGE(.BOTH.,#63903);
#63905=PRESENTATION_STYLE_ASSIGNMENT((#63904));
ENDSEC;
END-ISO-10303-21;
